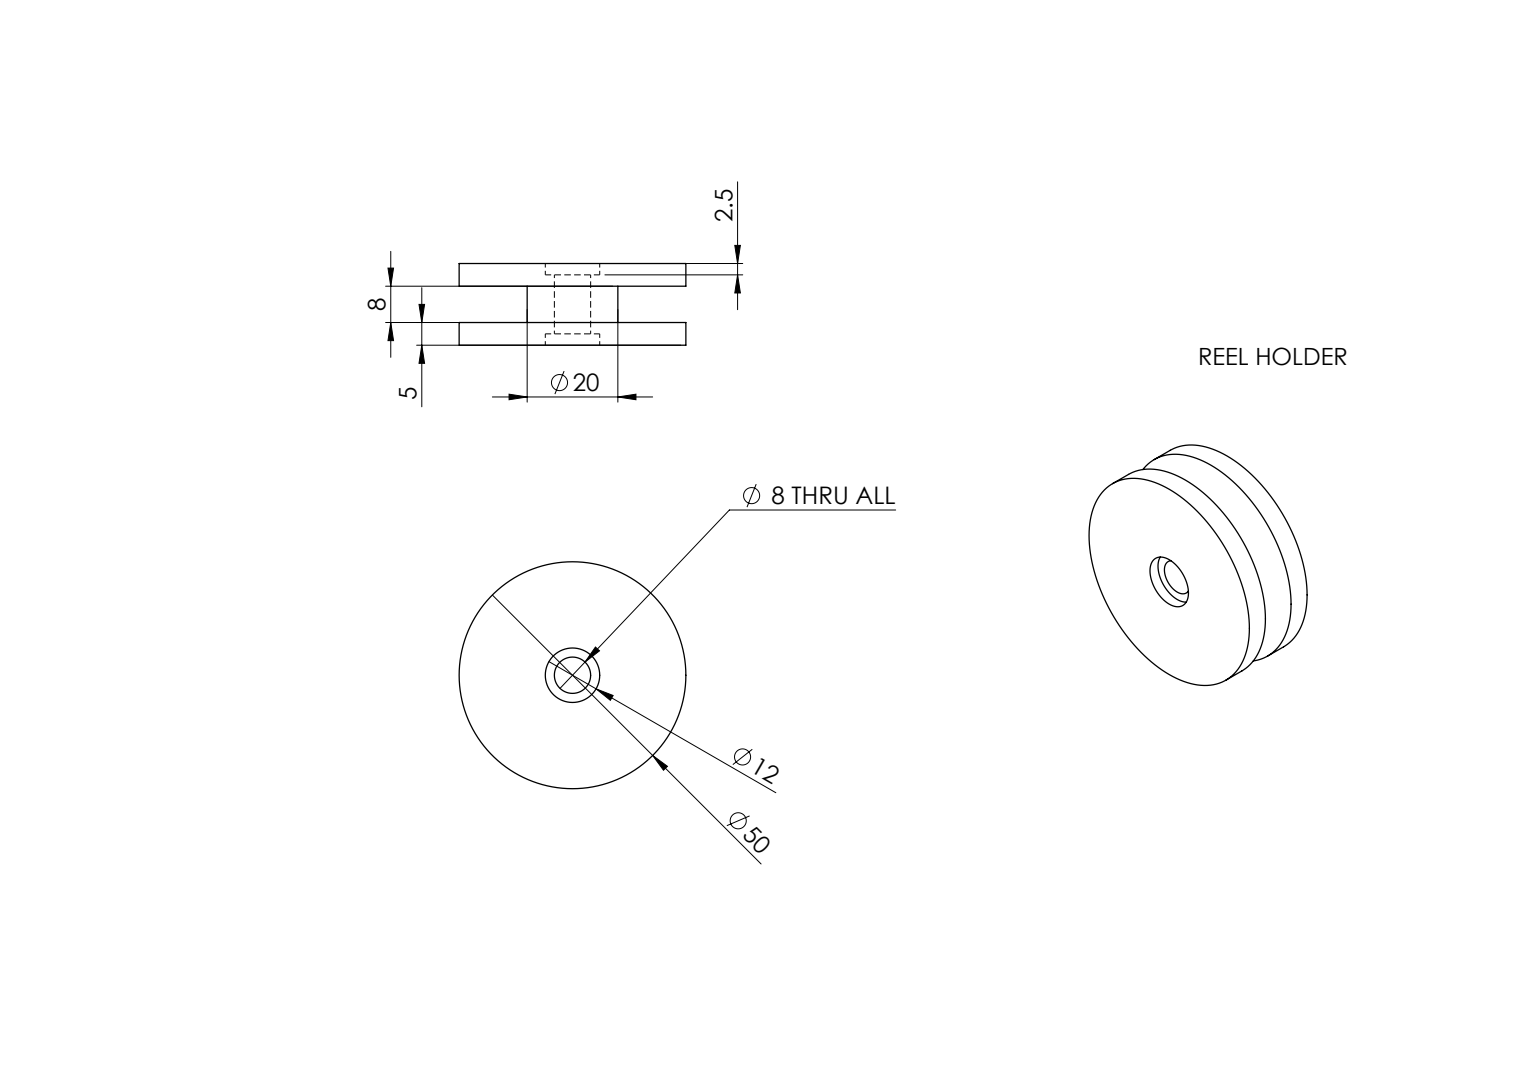
ISO-10303-21;
HEADER;
FILE_DESCRIPTION (('STEP AP214'),
    '1' );
FILE_NAME ('reel holder.step',
    '2026-10-31T03:44:21',
    ( '' ),
    ( '' ),
    'SwSTEP 2.0',
    'SolidWorks 2026',
    '' );
FILE_SCHEMA (( 'AUTOMOTIVE_DESIGN' ));
ENDSEC;

DATA;
#18=EDGE_LOOP ( 'NONE', ( #11625, #15008, #6307, #1224 ) ) ;
#22=AXIS2_PLACEMENT_3D ( 'NONE', #10156, #1151, #17072 ) ;
#37=( NAMED_UNIT ( * ) PLANE_ANGLE_UNIT ( ) SI_UNIT ( $, .RADIAN. ) );
#60=FACE_OUTER_BOUND ( 'NONE', #12914, .T. ) ;
#63=ADVANCED_FACE ( 'NONE', ( #9131 ), #4633, .F. ) ;
#64=ADVANCED_FACE ( 'NONE', ( #5901 ), #7658, .T. ) ;
#74=CIRCLE ( 'NONE', #18561, 24.99999999999999289 ) ;
#181=DIRECTION ( 'NONE',  ( 1.000000000000000000, 0.000000000000000000, 0.000000000000000000 ) ) ;
#266=CYLINDRICAL_SURFACE ( 'NONE', #9428, 5.999999999999977796 ) ;
#280=DIRECTION ( 'NONE',  ( 1.000000000000000000, 0.000000000000000000, 0.000000000000000000 ) ) ;
#318=ADVANCED_FACE ( 'NONE', ( #14500 ), #9696, .T. ) ;
#351=CARTESIAN_POINT ( 'NONE',  ( -154.9999999999999716, -14.99999999999999645, -6.499999999999999112 ) ) ;
#404=EDGE_CURVE ( 'NONE', #12345, #17767, #17395, .T. ) ;
#429=DIRECTION ( 'NONE',  ( -0.000000000000000000, -0.000000000000000000, 1.000000000000000000 ) ) ;
#448=ORIENTED_EDGE ( 'NONE', *, *, #5602, .F. ) ;
#586=CARTESIAN_POINT ( 'NONE',  ( -154.9999999999999716, -14.99999999999999645, 4.000000000000000000 ) ) ;
#587=CIRCLE ( 'NONE', #6229, 5.999999999999977796 ) ;
#601=VECTOR ( 'NONE', #10729, 1000.000000000000000 ) ;
#605=MECHANICAL_DESIGN_GEOMETRIC_PRESENTATION_REPRESENTATION('',(#15624),#12814);
#684=ORIENTED_EDGE ( 'NONE', *, *, #1869, .T. ) ;
#788=AXIS2_PLACEMENT_3D ( 'NONE', #11144, #17151, #5374 ) ;
#800=LINE ( 'NONE', #6771, #1505 ) ;
#861=DIRECTION ( 'NONE',  ( -1.000000000000000000, 0.000000000000000000, 0.000000000000000000 ) ) ;
#869=VERTEX_POINT ( 'NONE', #18994 ) ;
#870=VERTEX_POINT ( 'NONE', #11414 ) ;
#878=DIRECTION ( 'NONE',  ( -1.000000000000000000, 0.000000000000000000, 0.000000000000000000 ) ) ;
#884=DIRECTION ( 'NONE',  ( 1.000000000000000000, 0.000000000000000000, 0.000000000000000000 ) ) ;
#1016=ADVANCED_FACE ( 'NONE', ( #6034, #11998 ), #10619, .T. ) ;
#1038=PRODUCT_DEFINITION_FORMATION_WITH_SPECIFIED_SOURCE ( 'ANY', '', #17923, .NOT_KNOWN. ) ;
#1083=CARTESIAN_POINT ( 'NONE',  ( -154.9999999999999716, -14.99999999999999645, 4.000000000000000000 ) ) ;
#1151=DIRECTION ( 'NONE',  ( 0.000000000000000000, 0.000000000000000000, -1.000000000000000000 ) ) ;
#1224=ORIENTED_EDGE ( 'NONE', *, *, #8355, .F. ) ;
#1418=AXIS2_PLACEMENT_3D ( 'NONE', #5586, #3834, #884 ) ;
#1420=ORIENTED_EDGE ( 'NONE', *, *, #3761, .T. ) ;
#1439=EDGE_LOOP ( 'NONE', ( #2082, #16900, #12486, #14325 ) ) ;
#1454=EDGE_LOOP ( 'NONE', ( #9792, #2037 ) ) ;
#1483=PRODUCT_CONTEXT ( 'NONE', #11764, 'mechanical' ) ;
#1505=VECTOR ( 'NONE', #18753, 1000.000000000000000 ) ;
#1512=EDGE_LOOP ( 'NONE', ( #14590, #15562, #17642, #12838 ) ) ;
#1575=FACE_BOUND ( 'NONE', #7460, .T. ) ;
#1588=VECTOR ( 'NONE', #1817, 1000.000000000000000 ) ;
#1607=AXIS2_PLACEMENT_3D ( 'NONE', #1997, #7773, #4752 ) ;
#1609=PRESENTATION_STYLE_ASSIGNMENT (( #17632 ) ) ;
#1626=DIRECTION ( 'NONE',  ( 1.000000000000000000, 0.000000000000000000, 0.000000000000000000 ) ) ;
#1628=AXIS2_PLACEMENT_3D ( 'NONE', #3357, #15497, #5009 ) ;
#1636=ORIENTED_EDGE ( 'NONE', *, *, #8355, .T. ) ;
#1648=LINE ( 'NONE', #7515, #16648 ) ;
#1796=DIRECTION ( 'NONE',  ( -0.000000000000000000, -0.000000000000000000, 1.000000000000000000 ) ) ;
#1804=CARTESIAN_POINT ( 'NONE',  ( -179.9999999999999716, -15.00000000000000000, -9.000000000000000000 ) ) ;
#1817=DIRECTION ( 'NONE',  ( 0.000000000000000000, 0.000000000000000000, -1.000000000000000000 ) ) ;
#1835=( LENGTH_UNIT ( ) NAMED_UNIT ( * ) SI_UNIT ( .MILLI., .METRE. ) );
#1869=EDGE_CURVE ( 'NONE', #17340, #19190, #16799, .T. ) ;
#1997=CARTESIAN_POINT ( 'NONE',  ( -154.9999999999999716, -14.99999999999999645, -9.000000000000000000 ) ) ;
#2021=AXIS2_PLACEMENT_3D ( 'NONE', #12770, #10013, #11384 ) ;
#2037=ORIENTED_EDGE ( 'NONE', *, *, #13822, .F. ) ;
#2082=ORIENTED_EDGE ( 'NONE', *, *, #11418, .F. ) ;
#2102=CLOSED_SHELL ( 'NONE', ( #4793, #63, #16827, #318, #6766, #9044, #8811, #10108, #5089, #5235, #9436, #64, #16364, #16884, #4440, #2460, #1016, #18165 ) ) ;
#2171=( GEOMETRIC_REPRESENTATION_CONTEXT ( 3 ) GLOBAL_UNCERTAINTY_ASSIGNED_CONTEXT ( ( #4414 ) ) GLOBAL_UNIT_ASSIGNED_CONTEXT ( ( #11985, #15951, #16609 ) ) REPRESENTATION_CONTEXT ( 'NONE', 'WORKASPACE' ) );
#2173=CARTESIAN_POINT ( 'NONE',  ( -154.9999999999999716, -14.99999999999999645, 9.000000000000000000 ) ) ;
#2233=CIRCLE ( 'NONE', #4098, 5.999999999999977796 ) ;
#2309=ORIENTED_EDGE ( 'NONE', *, *, #9763, .F. ) ;
#2327=CIRCLE ( 'NONE', #4523, 24.99999999999999289 ) ;
#2420=VERTEX_POINT ( 'NONE', #9185 ) ;
#2460=ADVANCED_FACE ( 'NONE', ( #6430 ), #266, .F. ) ;
#2472=DIRECTION ( 'NONE',  ( -1.000000000000000000, 0.000000000000000000, 0.000000000000000000 ) ) ;
#2502=DIRECTION ( 'NONE',  ( 1.000000000000000000, 0.000000000000000000, -0.000000000000000000 ) ) ;
#2538=VERTEX_POINT ( 'NONE', #14440 ) ;
#2542=DIRECTION ( 'NONE',  ( 0.000000000000000000, 0.000000000000000000, 1.000000000000000000 ) ) ;
#2544=ORIENTED_EDGE ( 'NONE', *, *, #10861, .T. ) ;
#2576=CIRCLE ( 'NONE', #1628, 10.00000000000000888 ) ;
#2636=SURFACE_SIDE_STYLE ('',( #15030 ) ) ;
#2693=PLANE ( 'NONE',  #16419 ) ;
#2722=AXIS2_PLACEMENT_3D ( 'NONE', #2861, #11750, #13233 ) ;
#2816=EDGE_CURVE ( 'NONE', #19190, #17340, #74, .T. ) ;
#2861=CARTESIAN_POINT ( 'NONE',  ( -154.9999999999999716, -14.99999999999999645, 9.000000000000000000 ) ) ;
#2871=CARTESIAN_POINT ( 'NONE',  ( 0.000000000000000000, 0.000000000000000000, 0.000000000000000000 ) ) ;
#2872=EDGE_CURVE ( 'NONE', #7670, #17070, #14138, .T. ) ;
#2989=CARTESIAN_POINT ( 'NONE',  ( -154.9999999999999716, -14.99999999999999645, -9.000000000000000000 ) ) ;
#3030=VERTEX_POINT ( 'NONE', #7423 ) ;
#3069=AXIS2_PLACEMENT_3D ( 'NONE', #10990, #3551, #16996 ) ;
#3073=STYLED_ITEM('',(#19461),#8428);
#3119=CARTESIAN_POINT ( 'NONE',  ( -160.9999999999999432, -14.99999999999999645, -6.499999999999999112 ) ) ;
#3161=CIRCLE ( 'NONE', #10321, 4.000000000000003553 ) ;
#3180=CIRCLE ( 'NONE', #1607, 5.999999999999977796 ) ;
#3357=CARTESIAN_POINT ( 'NONE',  ( -154.9999999999999716, -14.99999999999999645, 4.000000000000000000 ) ) ;
#3366=CARTESIAN_POINT ( 'NONE',  ( -158.9999999999999716, -14.99999999999999645, 15.00000000000000000 ) ) ;
#3393=VERTEX_POINT ( 'NONE', #6121 ) ;
#3476=PLANE ( 'NONE',  #12019 ) ;
#3551=DIRECTION ( 'NONE',  ( -0.000000000000000000, -0.000000000000000000, 1.000000000000000000 ) ) ;
#3652=LINE ( 'NONE', #3366, #18836 ) ;
#3761=EDGE_CURVE ( 'NONE', #17070, #7670, #11391, .T. ) ;
#3792=EDGE_CURVE ( 'NONE', #8294, #12345, #18966, .T. ) ;
#3834=DIRECTION ( 'NONE',  ( -0.000000000000000000, -0.000000000000000000, 1.000000000000000000 ) ) ;
#3923=VERTEX_POINT ( 'NONE', #7566 ) ;
#3952=CARTESIAN_POINT ( 'NONE',  ( -129.9999999999999716, -14.99999999999999645, -3.999999999999999112 ) ) ;
#4000=CIRCLE ( 'NONE', #12439, 4.000000000000003553 ) ;
#4005=CARTESIAN_POINT ( 'NONE',  ( -160.9999999999999432, -14.99999999999999645, 9.000000000000000000 ) ) ;
#4010=ORIENTED_EDGE ( 'NONE', *, *, #7307, .F. ) ;
#4018=EDGE_CURVE ( 'NONE', #4718, #4669, #18635, .T. ) ;
#4042=DIRECTION ( 'NONE',  ( 1.000000000000000000, 0.000000000000000000, 0.000000000000000000 ) ) ;
#4098=AXIS2_PLACEMENT_3D ( 'NONE', #2989, #16516, #5825 ) ;
#4160=DIRECTION ( 'NONE',  ( 1.000000000000000000, 0.000000000000000000, 0.000000000000000000 ) ) ;
#4180=DIRECTION ( 'NONE',  ( 1.000000000000000000, 0.000000000000000000, 0.000000000000000000 ) ) ;
#4185=ORIENTED_EDGE ( 'NONE', *, *, #6921, .T. ) ;
#4252=ORIENTED_EDGE ( 'NONE', *, *, #5602, .T. ) ;
#4344=ORIENTED_EDGE ( 'NONE', *, *, #14162, .F. ) ;
#4374=CIRCLE ( 'NONE', #15323, 4.000000000000003553 ) ;
#4414=UNCERTAINTY_MEASURE_WITH_UNIT (LENGTH_MEASURE( 1.000000000000000082E-05 ), #11985, 'distance_accuracy_value', 'NONE');
#4428=DIRECTION ( 'NONE',  ( 0.000000000000000000, 0.000000000000000000, -1.000000000000000000 ) ) ;
#4429=CARTESIAN_POINT ( 'NONE',  ( -150.9999999999999716, -14.99999999999999645, 15.00000000000000000 ) ) ;
#4437=FACE_OUTER_BOUND ( 'NONE', #17799, .T. ) ;
#4440=ADVANCED_FACE ( 'NONE', ( #19342, #1575 ), #5884, .T. ) ;
#4474=ORIENTED_EDGE ( 'NONE', *, *, #13822, .T. ) ;
#4475=DIRECTION ( 'NONE',  ( 0.000000000000000000, 0.000000000000000000, 1.000000000000000000 ) ) ;
#4495=CARTESIAN_POINT ( 'NONE',  ( -129.9999999999999716, -14.99999999999999645, -3.999999999999999112 ) ) ;
#4523=AXIS2_PLACEMENT_3D ( 'NONE', #13255, #9818, #8558 ) ;
#4534=AXIS2_PLACEMENT_3D ( 'NONE', #2173, #15305, #18460 ) ;
#4562=DIRECTION ( 'NONE',  ( 0.000000000000000000, 0.000000000000000000, -1.000000000000000000 ) ) ;
#4563=DIRECTION ( 'NONE',  ( -0.000000000000000000, -0.000000000000000000, 1.000000000000000000 ) ) ;
#4567=CARTESIAN_POINT ( 'NONE',  ( -179.9999999999999716, -14.99999999999999289, 3.999999999999999112 ) ) ;
#4633=CYLINDRICAL_SURFACE ( 'NONE', #16829, 5.999999999999977796 ) ;
#4669=VERTEX_POINT ( 'NONE', #4005 ) ;
#4689=( NAMED_UNIT ( * ) SI_UNIT ( $, .STERADIAN. ) SOLID_ANGLE_UNIT ( ) );
#4703=AXIS2_PLACEMENT_3D ( 'NONE', #16401, #14611, #4042 ) ;
#4718=VERTEX_POINT ( 'NONE', #5273 ) ;
#4752=DIRECTION ( 'NONE',  ( 1.000000000000000000, 0.000000000000000000, 0.000000000000000000 ) ) ;
#4755=DIRECTION ( 'NONE',  ( 0.000000000000000000, 0.000000000000000000, -1.000000000000000000 ) ) ;
#4759=FACE_OUTER_BOUND ( 'NONE', #18, .T. ) ;
#4783=DIRECTION ( 'NONE',  ( 1.000000000000000000, 0.000000000000000000, 0.000000000000000000 ) ) ;
#4793=ADVANCED_FACE ( 'NONE', ( #11346 ), #5172, .F. ) ;
#4852=DIRECTION ( 'NONE',  ( -0.000000000000000000, -0.000000000000000000, 1.000000000000000000 ) ) ;
#4874=CARTESIAN_POINT ( 'NONE',  ( -154.9999999999999716, -14.99999999999999645, 6.499999999999999112 ) ) ;
#4952=VERTEX_POINT ( 'NONE', #19224 ) ;
#4966=CIRCLE ( 'NONE', #10293, 10.00000000000000888 ) ;
#5009=DIRECTION ( 'NONE',  ( 1.000000000000000000, 0.000000000000000000, 0.000000000000000000 ) ) ;
#5089=ADVANCED_FACE ( 'NONE', ( #6691, #12773 ), #3476, .F. ) ;
#5172=CYLINDRICAL_SURFACE ( 'NONE', #788, 5.999999999999977796 ) ;
#5216=AXIS2_PLACEMENT_3D ( 'NONE', #18382, #429, #10898 ) ;
#5235=ADVANCED_FACE ( 'NONE', ( #19271, #5510 ), #2693, .T. ) ;
#5254=ORIENTED_EDGE ( 'NONE', *, *, #5301, .T. ) ;
#5262=CARTESIAN_POINT ( 'NONE',  ( -154.9999999999999716, -14.99999999999999645, 9.000000000000000000 ) ) ;
#5273=CARTESIAN_POINT ( 'NONE',  ( -149.0000000000000000, -14.99999999999999645, 9.000000000000000000 ) ) ;
#5298=CIRCLE ( 'NONE', #6245, 5.999999999999977796 ) ;
#5301=EDGE_CURVE ( 'NONE', #16254, #8294, #2327, .T. ) ;
#5313=CARTESIAN_POINT ( 'NONE',  ( -129.9999999999999716, -14.99999999999999645, -9.000000000000000000 ) ) ;
#5320=DIRECTION ( 'NONE',  ( 1.000000000000000000, 0.000000000000000000, -0.000000000000000000 ) ) ;
#5374=DIRECTION ( 'NONE',  ( 1.000000000000000000, 0.000000000000000000, 0.000000000000000000 ) ) ;
#5510=FACE_OUTER_BOUND ( 'NONE', #8020, .T. ) ;
#5545=EDGE_CURVE ( 'NONE', #869, #3393, #10306, .T. ) ;
#5586=CARTESIAN_POINT ( 'NONE',  ( -154.9999999999999716, -14.99999999999999645, -9.000000000000000000 ) ) ;
#5602=EDGE_CURVE ( 'NONE', #869, #10775, #2576, .T. ) ;
#5647=CARTESIAN_POINT ( 'NONE',  ( -154.9999999999999716, -14.99999999999999645, 6.499999999999999112 ) ) ;
#5655=FACE_OUTER_BOUND ( 'NONE', #5723, .T. ) ;
#5661=DIRECTION ( 'NONE',  ( 1.000000000000000000, 0.000000000000000000, 0.000000000000000000 ) ) ;
#5675=AXIS2_PLACEMENT_3D ( 'NONE', #10237, #12002, #16238 ) ;
#5706=DIRECTION ( 'NONE',  ( 1.000000000000000000, 0.000000000000000000, 0.000000000000000000 ) ) ;
#5710=FACE_BOUND ( 'NONE', #1454, .T. ) ;
#5723=EDGE_LOOP ( 'NONE', ( #14570, #18536, #6745, #15319 ) ) ;
#5782=UNCERTAINTY_MEASURE_WITH_UNIT (LENGTH_MEASURE( 1.000000000000000082E-05 ), #1835, 'distance_accuracy_value', 'NONE');
#5825=DIRECTION ( 'NONE',  ( 1.000000000000000000, 0.000000000000000000, 0.000000000000000000 ) ) ;
#5864=EDGE_LOOP ( 'NONE', ( #9344, #6932, #10169, #7931 ) ) ;
#5884=PLANE ( 'NONE',  #10782 ) ;
#5901=FACE_OUTER_BOUND ( 'NONE', #18988, .T. ) ;
#5998=VECTOR ( 'NONE', #19401, 1000.000000000000000 ) ;
#6034=FACE_OUTER_BOUND ( 'NONE', #9664, .T. ) ;
#6113=CIRCLE ( 'NONE', #11103, 10.00000000000000888 ) ;
#6121=CARTESIAN_POINT ( 'NONE',  ( -144.9999999999999716, -14.99999999999999467, -4.000000000000000000 ) ) ;
#6229=AXIS2_PLACEMENT_3D ( 'NONE', #5262, #2542, #8204 ) ;
#6238=ORIENTED_EDGE ( 'NONE', *, *, #17697, .T. ) ;
#6245=AXIS2_PLACEMENT_3D ( 'NONE', #5647, #4475, #4180 ) ;
#6251=DIRECTION ( 'NONE',  ( 0.000000000000000000, 0.000000000000000000, 1.000000000000000000 ) ) ;
#6264=PRODUCT_DEFINITION ( 'UNKNOWN', '', #1038, #9291 ) ;
#6307=ORIENTED_EDGE ( 'NONE', *, *, #7307, .T. ) ;
#6428=DIRECTION ( 'NONE',  ( 1.000000000000000000, 0.000000000000000000, 0.000000000000000000 ) ) ;
#6430=FACE_OUTER_BOUND ( 'NONE', #16684, .T. ) ;
#6436=AXIS2_PLACEMENT_3D ( 'NONE', #12043, #7630, #280 ) ;
#6458=ORIENTED_EDGE ( 'NONE', *, *, #404, .F. ) ;
#6481=VECTOR ( 'NONE', #6846, 1000.000000000000000 ) ;
#6500=DIRECTION ( 'NONE',  ( -1.000000000000000000, 0.000000000000000000, 0.000000000000000000 ) ) ;
#6560=FACE_OUTER_BOUND ( 'NONE', #1512, .T. ) ;
#6662=DIRECTION ( 'NONE',  ( -0.000000000000000000, -0.000000000000000000, -1.000000000000000000 ) ) ;
#6691=FACE_BOUND ( 'NONE', #6831, .T. ) ;
#6745=ORIENTED_EDGE ( 'NONE', *, *, #19262, .T. ) ;
#6755=DIRECTION ( 'NONE',  ( 1.000000000000000000, 0.000000000000000000, 0.000000000000000000 ) ) ;
#6766=ADVANCED_FACE ( 'NONE', ( #60 ), #17714, .T. ) ;
#6771=CARTESIAN_POINT ( 'NONE',  ( -164.9999999999999716, -14.99999999999999645, 4.000000000000000000 ) ) ;
#6805=ORIENTED_EDGE ( 'NONE', *, *, #9511, .T. ) ;
#6831=EDGE_LOOP ( 'NONE', ( #15973, #4252 ) ) ;
#6846=DIRECTION ( 'NONE',  ( -0.000000000000000000, -0.000000000000000000, 1.000000000000000000 ) ) ;
#6921=EDGE_CURVE ( 'NONE', #7670, #19190, #13379, .T. ) ;
#6932=ORIENTED_EDGE ( 'NONE', *, *, #2872, .T. ) ;
#7024=ORIENTED_EDGE ( 'NONE', *, *, #9763, .T. ) ;
#7170=CARTESIAN_POINT ( 'NONE',  ( -154.9999999999999716, -14.99999999999999645, 4.000000000000000000 ) ) ;
#7187=VERTEX_POINT ( 'NONE', #11487 ) ;
#7190=ORIENTED_EDGE ( 'NONE', *, *, #3761, .F. ) ;
#7213=AXIS2_PLACEMENT_3D ( 'NONE', #13647, #1796, #14017 ) ;
#7298=ORIENTED_EDGE ( 'NONE', *, *, #15386, .T. ) ;
#7307=EDGE_CURVE ( 'NONE', #7187, #9732, #14906, .T. ) ;
#7355=AXIS2_PLACEMENT_3D ( 'NONE', #10428, #4563, #16718 ) ;
#7365=AXIS2_PLACEMENT_3D ( 'NONE', #1083, #12649, #2472 ) ;
#7423=CARTESIAN_POINT ( 'NONE',  ( -160.9999999999999432, -14.99999999999999645, -9.000000000000000000 ) ) ;
#7434=ORIENTED_EDGE ( 'NONE', *, *, #12646, .F. ) ;
#7440=( GEOMETRIC_REPRESENTATION_CONTEXT ( 3 ) GLOBAL_UNCERTAINTY_ASSIGNED_CONTEXT ( ( #5782 ) ) GLOBAL_UNIT_ASSIGNED_CONTEXT ( ( #1835, #18126, #4689 ) ) REPRESENTATION_CONTEXT ( 'NONE', 'WORKASPACE' ) );
#7460=EDGE_LOOP ( 'NONE', ( #11837, #1636 ) ) ;
#7486=EDGE_CURVE ( 'NONE', #2420, #11109, #13567, .T. ) ;
#7515=CARTESIAN_POINT ( 'NONE',  ( -160.9999999999999432, -14.99999999999999645, -6.499999999999999112 ) ) ;
#7564=CARTESIAN_POINT ( 'NONE',  ( -129.9999999999999716, -14.99999999999999645, 3.999999999999999112 ) ) ;
#7566=CARTESIAN_POINT ( 'NONE',  ( -149.0000000000000000, -14.99999999999999645, 6.499999999999999112 ) ) ;
#7576=( LENGTH_UNIT ( ) NAMED_UNIT ( * ) SI_UNIT ( .MILLI., .METRE. ) );
#7598=EDGE_CURVE ( 'NONE', #8294, #16254, #8336, .T. ) ;
#7613=DIRECTION ( 'NONE',  ( 1.000000000000000000, 0.000000000000000000, 0.000000000000000000 ) ) ;
#7630=DIRECTION ( 'NONE',  ( -0.000000000000000000, -0.000000000000000000, 1.000000000000000000 ) ) ;
#7658=CYLINDRICAL_SURFACE ( 'NONE', #13051, 24.99999999999999289 ) ;
#7670=VERTEX_POINT ( 'NONE', #11187 ) ;
#7773=DIRECTION ( 'NONE',  ( -0.000000000000000000, -0.000000000000000000, 1.000000000000000000 ) ) ;
#7931=ORIENTED_EDGE ( 'NONE', *, *, #2816, .F. ) ;
#7953=VECTOR ( 'NONE', #15911, 1000.000000000000000 ) ;
#8020=EDGE_LOOP ( 'NONE', ( #684, #16341 ) ) ;
#8132=DIRECTION ( 'NONE',  ( 0.000000000000000000, 0.000000000000000000, 1.000000000000000000 ) ) ;
#8204=DIRECTION ( 'NONE',  ( 1.000000000000000000, 0.000000000000000000, 0.000000000000000000 ) ) ;
#8226=CARTESIAN_POINT ( 'NONE',  ( -154.9999999999999716, -14.99999999999999645, -9.000000000000000000 ) ) ;
#8294=VERTEX_POINT ( 'NONE', #4495 ) ;
#8319=CARTESIAN_POINT ( 'NONE',  ( -154.9999999999999716, -14.99999999999999645, 6.499999999999999112 ) ) ;
#8336=CIRCLE ( 'NONE', #5216, 24.99999999999999289 ) ;
#8355=EDGE_CURVE ( 'NONE', #4952, #9732, #4000, .T. ) ;
#8394=DIRECTION ( 'NONE',  ( 1.000000000000000000, 0.000000000000000000, 0.000000000000000000 ) ) ;
#8428=MANIFOLD_SOLID_BREP ( 'Mirror3', #2102 ) ;
#8503=ORIENTED_EDGE ( 'NONE', *, *, #18760, .F. ) ;
#8558=DIRECTION ( 'NONE',  ( 1.000000000000000000, 0.000000000000000000, 0.000000000000000000 ) ) ;
#8589=FILL_AREA_STYLE ('',( #9041 ) ) ;
#8595=CARTESIAN_POINT ( 'NONE',  ( -154.9999999999999716, -14.99999999999999645, 3.999999999999999112 ) ) ;
#8665=SHAPE_REPRESENTATION ( 'reel holder', ( #10359 ), #2171 ) ;
#8794=ORIENTED_EDGE ( 'NONE', *, *, #2872, .F. ) ;
#8811=ADVANCED_FACE ( 'NONE', ( #4759 ), #10720, .F. ) ;
#8834=DIRECTION ( 'NONE',  ( 0.000000000000000000, 0.000000000000000000, 1.000000000000000000 ) ) ;
#8842=DIRECTION ( 'NONE',  ( -0.000000000000000000, -0.000000000000000000, 1.000000000000000000 ) ) ;
#8856=DIRECTION ( 'NONE',  ( -0.000000000000000000, -0.000000000000000000, -1.000000000000000000 ) ) ;
#8996=CIRCLE ( 'NONE', #3069, 5.999999999999977796 ) ;
#9017=SHAPE_DEFINITION_REPRESENTATION ( #19343, #8665 ) ;
#9041=FILL_AREA_STYLE_COLOUR ( '', #17203 ) ;
#9044=ADVANCED_FACE ( 'NONE', ( #17185 ), #17383, .F. ) ;
#9113=DIRECTION ( 'NONE',  ( 1.000000000000000000, 0.000000000000000000, -0.000000000000000000 ) ) ;
#9131=FACE_OUTER_BOUND ( 'NONE', #15370, .T. ) ;
#9148=EDGE_CURVE ( 'NONE', #10775, #869, #6113, .T. ) ;
#9170=CARTESIAN_POINT ( 'NONE',  ( -154.9999999999999716, -14.99999999999999645, 15.00000000000000000 ) ) ;
#9185=CARTESIAN_POINT ( 'NONE',  ( -149.0000000000000000, -14.99999999999999645, -6.499999999999999112 ) ) ;
#9223=CARTESIAN_POINT ( 'NONE',  ( -144.9999999999999716, -14.99999999999999467, 4.000000000000000000 ) ) ;
#9291=PRODUCT_DEFINITION_CONTEXT ( 'detailed design', #18441, 'design' ) ;
#9344=ORIENTED_EDGE ( 'NONE', *, *, #6921, .F. ) ;
#9428=AXIS2_PLACEMENT_3D ( 'NONE', #13786, #12222, #4783 ) ;
#9436=ADVANCED_FACE ( 'NONE', ( #6560 ), #15586, .T. ) ;
#9494=ORIENTED_EDGE ( 'NONE', *, *, #404, .T. ) ;
#9511=EDGE_CURVE ( 'NONE', #3923, #2538, #10182, .T. ) ;
#9575=DIRECTION ( 'NONE',  ( -0.000000000000000000, -0.000000000000000000, 1.000000000000000000 ) ) ;
#9608=DIRECTION ( 'NONE',  ( 1.000000000000000000, 0.000000000000000000, 0.000000000000000000 ) ) ;
#9659=CIRCLE ( 'NONE', #14677, 10.00000000000000888 ) ;
#9664=EDGE_LOOP ( 'NONE', ( #2309, #7434 ) ) ;
#9691=FACE_BOUND ( 'NONE', #11497, .T. ) ;
#9696=CYLINDRICAL_SURFACE ( 'NONE', #7365, 10.00000000000000888 ) ;
#9724=CARTESIAN_POINT ( 'NONE',  ( -154.9999999999999716, -14.99999999999999645, 3.999999999999999112 ) ) ;
#9732=VERTEX_POINT ( 'NONE', #16082 ) ;
#9736=EDGE_LOOP ( 'NONE', ( #7190, #8794 ) ) ;
#9763=EDGE_CURVE ( 'NONE', #2420, #11339, #16784, .T. ) ;
#9792=ORIENTED_EDGE ( 'NONE', *, *, #13722, .F. ) ;
#9818=DIRECTION ( 'NONE',  ( -0.000000000000000000, -0.000000000000000000, 1.000000000000000000 ) ) ;
#9917=DIRECTION ( 'NONE',  ( 0.000000000000000000, 0.000000000000000000, 1.000000000000000000 ) ) ;
#9999=LINE ( 'NONE', #19156, #12829 ) ;
#10013=DIRECTION ( 'NONE',  ( 0.000000000000000000, 0.000000000000000000, 1.000000000000000000 ) ) ;
#10033=CARTESIAN_POINT ( 'NONE',  ( -164.9999999999999716, -14.99999999999999645, 4.000000000000000000 ) ) ;
#10037=EDGE_LOOP ( 'NONE', ( #7024, #15755, #16509, #14469 ) ) ;
#10076=AXIS2_PLACEMENT_3D ( 'NONE', #13299, #15251, #7613 ) ;
#10108=ADVANCED_FACE ( 'NONE', ( #14272 ), #17535, .T. ) ;
#10155=DIRECTION ( 'NONE',  ( 0.000000000000000000, 0.000000000000000000, 1.000000000000000000 ) ) ;
#10156=CARTESIAN_POINT ( 'NONE',  ( -154.9999999999999716, -14.99999999999999645, -3.999999999999999112 ) ) ;
#10169=ORIENTED_EDGE ( 'NONE', *, *, #18097, .T. ) ;
#10182=CIRCLE ( 'NONE', #18976, 5.999999999999977796 ) ;
#10237=CARTESIAN_POINT ( 'NONE',  ( -154.9999999999999716, -14.99999999999999645, 3.999999999999999112 ) ) ;
#10293=AXIS2_PLACEMENT_3D ( 'NONE', #13972, #15457, #13880 ) ;
#10306=LINE ( 'NONE', #9223, #11942 ) ;
#10321=AXIS2_PLACEMENT_3D ( 'NONE', #351, #4852, #6500 ) ;
#10330=AXIS2_PLACEMENT_3D ( 'NONE', #8226, #15485, #6755 ) ;
#10359=AXIS2_PLACEMENT_3D ( 'NONE', #2871, #8834, #16191 ) ;
#10401=PLANE ( 'NONE',  #4703 ) ;
#10417=CARTESIAN_POINT ( 'NONE',  ( -164.9999999999999716, -14.99999999999999645, -4.000000000000000000 ) ) ;
#10428=CARTESIAN_POINT ( 'NONE',  ( -154.9999999999999716, -14.99999999999999645, 15.00000000000000000 ) ) ;
#10490=ORIENTED_EDGE ( 'NONE', *, *, #12984, .F. ) ;
#10529=LINE ( 'NONE', #13859, #601 ) ;
#10619=PLANE ( 'NONE',  #13081 ) ;
#10720=CYLINDRICAL_SURFACE ( 'NONE', #7355, 4.000000000000003553 ) ;
#10729=DIRECTION ( 'NONE',  ( -0.000000000000000000, -0.000000000000000000, 1.000000000000000000 ) ) ;
#10733=ORIENTED_EDGE ( 'NONE', *, *, #17722, .T. ) ;
#10775=VERTEX_POINT ( 'NONE', #10033 ) ;
#10782=AXIS2_PLACEMENT_3D ( 'NONE', #16386, #11851, #9113 ) ;
#10861=EDGE_CURVE ( 'NONE', #3030, #11109, #2233, .T. ) ;
#10898=DIRECTION ( 'NONE',  ( 1.000000000000000000, 0.000000000000000000, 0.000000000000000000 ) ) ;
#10951=CARTESIAN_POINT ( 'NONE',  ( -149.0000000000000000, -14.99999999999999645, -9.000000000000000000 ) ) ;
#10990=CARTESIAN_POINT ( 'NONE',  ( -154.9999999999999716, -14.99999999999999645, -6.499999999999999112 ) ) ;
#10992=EDGE_CURVE ( 'NONE', #870, #4952, #3652, .T. ) ;
#10997=DIRECTION ( 'NONE',  ( -0.000000000000000000, -0.000000000000000000, 1.000000000000000000 ) ) ;
#11103=AXIS2_PLACEMENT_3D ( 'NONE', #7170, #17587, #5706 ) ;
#11109=VERTEX_POINT ( 'NONE', #10951 ) ;
#11144=CARTESIAN_POINT ( 'NONE',  ( -154.9999999999999716, -14.99999999999999645, -6.499999999999999112 ) ) ;
#11187=CARTESIAN_POINT ( 'NONE',  ( -179.9999999999999716, -14.99999999999999289, 3.999999999999999112 ) ) ;
#11339=VERTEX_POINT ( 'NONE', #3119 ) ;
#11346=FACE_OUTER_BOUND ( 'NONE', #10037, .T. ) ;
#11384=DIRECTION ( 'NONE',  ( 1.000000000000000000, 0.000000000000000000, 0.000000000000000000 ) ) ;
#11391=CIRCLE ( 'NONE', #2021, 24.99999999999999289 ) ;
#11414=CARTESIAN_POINT ( 'NONE',  ( -158.9999999999999716, -14.99999999999999645, -6.499999999999999112 ) ) ;
#11418=EDGE_CURVE ( 'NONE', #11339, #3030, #1648, .T. ) ;
#11487=CARTESIAN_POINT ( 'NONE',  ( -150.9999999999999716, -14.99999999999999645, -6.499999999999999112 ) ) ;
#11497=EDGE_LOOP ( 'NONE', ( #10733, #2544 ) ) ;
#11548=ORIENTED_EDGE ( 'NONE', *, *, #4018, .T. ) ;
#11607=AXIS2_PLACEMENT_3D ( 'NONE', #18340, #9575, #861 ) ;
#11625=ORIENTED_EDGE ( 'NONE', *, *, #10992, .F. ) ;
#11750=DIRECTION ( 'NONE',  ( 0.000000000000000000, 0.000000000000000000, 1.000000000000000000 ) ) ;
#11764=APPLICATION_CONTEXT ( 'automotive_design' ) ;
#11837=ORIENTED_EDGE ( 'NONE', *, *, #14592, .T. ) ;
#11851=DIRECTION ( 'NONE',  ( 0.000000000000000000, 0.000000000000000000, 1.000000000000000000 ) ) ;
#11857=CARTESIAN_POINT ( 'NONE',  ( -154.9999999999999716, -14.99999999999999645, -6.499999999999999112 ) ) ;
#11942=VECTOR ( 'NONE', #16313, 1000.000000000000000 ) ;
#11974=CARTESIAN_POINT ( 'NONE',  ( -154.9999999999999716, -14.99999999999999645, 6.499999999999999112 ) ) ;
#11985=( LENGTH_UNIT ( ) NAMED_UNIT ( * ) SI_UNIT ( .MILLI., .METRE. ) );
#11998=FACE_BOUND ( 'NONE', #13148, .T. ) ;
#12002=DIRECTION ( 'NONE',  ( 0.000000000000000000, 0.000000000000000000, 1.000000000000000000 ) ) ;
#12005=ORIENTED_EDGE ( 'NONE', *, *, #12504, .F. ) ;
#12016=DIRECTION ( 'NONE',  ( 0.000000000000000000, 0.000000000000000000, -1.000000000000000000 ) ) ;
#12019=AXIS2_PLACEMENT_3D ( 'NONE', #9724, #18775, #5320 ) ;
#12043=CARTESIAN_POINT ( 'NONE',  ( -154.9999999999999716, -14.99999999999999645, -6.499999999999999112 ) ) ;
#12197=LINE ( 'NONE', #13667, #1588 ) ;
#12222=DIRECTION ( 'NONE',  ( -0.000000000000000000, -0.000000000000000000, 1.000000000000000000 ) ) ;
#12345=VERTEX_POINT ( 'NONE', #5313 ) ;
#12439=AXIS2_PLACEMENT_3D ( 'NONE', #4874, #16552, #6428 ) ;
#12486=ORIENTED_EDGE ( 'NONE', *, *, #7486, .T. ) ;
#12504=EDGE_CURVE ( 'NONE', #2538, #4669, #18935, .T. ) ;
#12546=DIRECTION ( 'NONE',  ( 1.000000000000000000, 0.000000000000000000, 0.000000000000000000 ) ) ;
#12646=EDGE_CURVE ( 'NONE', #11339, #2420, #8996, .T. ) ;
#12649=DIRECTION ( 'NONE',  ( -0.000000000000000000, -0.000000000000000000, -1.000000000000000000 ) ) ;
#12770=CARTESIAN_POINT ( 'NONE',  ( -154.9999999999999716, -14.99999999999999645, 3.999999999999999112 ) ) ;
#12773=FACE_OUTER_BOUND ( 'NONE', #9736, .T. ) ;
#12814=( GEOMETRIC_REPRESENTATION_CONTEXT ( 3 ) GLOBAL_UNCERTAINTY_ASSIGNED_CONTEXT ( ( #16573 ) ) GLOBAL_UNIT_ASSIGNED_CONTEXT ( ( #7576, #37, #13558 ) ) REPRESENTATION_CONTEXT ( 'NONE', 'WORKASPACE' ) );
#12829=VECTOR ( 'NONE', #15997, 1000.000000000000000 ) ;
#12838=ORIENTED_EDGE ( 'NONE', *, *, #13722, .T. ) ;
#12914=EDGE_LOOP ( 'NONE', ( #1420, #4185, #13658, #17271 ) ) ;
#12961=CARTESIAN_POINT ( 'NONE',  ( -154.9999999999999716, -14.99999999999999645, 9.000000000000000000 ) ) ;
#12984=EDGE_CURVE ( 'NONE', #10775, #16015, #800, .T. ) ;
#13044=CYLINDRICAL_SURFACE ( 'NONE', #16283, 5.999999999999977796 ) ;
#13051=AXIS2_PLACEMENT_3D ( 'NONE', #13638, #17978, #19266 ) ;
#13081=AXIS2_PLACEMENT_3D ( 'NONE', #18002, #4562, #1626 ) ;
#13104=FACE_OUTER_BOUND ( 'NONE', #15291, .T. ) ;
#13148=EDGE_LOOP ( 'NONE', ( #19416, #6238 ) ) ;
#13233=DIRECTION ( 'NONE',  ( 1.000000000000000000, 0.000000000000000000, 0.000000000000000000 ) ) ;
#13255=CARTESIAN_POINT ( 'NONE',  ( -154.9999999999999716, -14.99999999999999645, -3.999999999999999112 ) ) ;
#13286=ORIENTED_EDGE ( 'NONE', *, *, #7598, .T. ) ;
#13299=CARTESIAN_POINT ( 'NONE',  ( -154.9999999999999716, -14.99999999999999645, 3.999999999999999112 ) ) ;
#13379=LINE ( 'NONE', #4567, #5998 ) ;
#13558=( NAMED_UNIT ( * ) SI_UNIT ( $, .STERADIAN. ) SOLID_ANGLE_UNIT ( ) );
#13567=LINE ( 'NONE', #18095, #13968 ) ;
#13638=CARTESIAN_POINT ( 'NONE',  ( -154.9999999999999716, -14.99999999999999645, -3.999999999999999112 ) ) ;
#13647=CARTESIAN_POINT ( 'NONE',  ( -154.9999999999999716, -14.99999999999999645, -9.000000000000000000 ) ) ;
#13658=ORIENTED_EDGE ( 'NONE', *, *, #1869, .F. ) ;
#13667=CARTESIAN_POINT ( 'NONE',  ( -179.9999999999999716, -15.00000000000000000, -3.999999999999999112 ) ) ;
#13722=EDGE_CURVE ( 'NONE', #16015, #3393, #4966, .T. ) ;
#13786=CARTESIAN_POINT ( 'NONE',  ( -154.9999999999999716, -14.99999999999999645, 6.499999999999999112 ) ) ;
#13799=EDGE_LOOP ( 'NONE', ( #448, #19384, #4474, #10490 ) ) ;
#13822=EDGE_CURVE ( 'NONE', #3393, #16015, #9659, .T. ) ;
#13859=CARTESIAN_POINT ( 'NONE',  ( -149.0000000000000000, -14.99999999999999645, 6.499999999999999112 ) ) ;
#13880=DIRECTION ( 'NONE',  ( 1.000000000000000000, 0.000000000000000000, 0.000000000000000000 ) ) ;
#13900=EDGE_LOOP ( 'NONE', ( #18381, #15247 ) ) ;
#13968=VECTOR ( 'NONE', #4755, 1000.000000000000000 ) ;
#13972=CARTESIAN_POINT ( 'NONE',  ( -154.9999999999999716, -14.99999999999999645, -4.000000000000000000 ) ) ;
#14017=DIRECTION ( 'NONE',  ( 1.000000000000000000, 0.000000000000000000, 0.000000000000000000 ) ) ;
#14023=CARTESIAN_POINT ( 'NONE',  ( -179.9999999999999716, -15.00000000000000000, -3.999999999999999112 ) ) ;
#14106=CIRCLE ( 'NONE', #11607, 4.000000000000003553 ) ;
#14138=CIRCLE ( 'NONE', #10076, 24.99999999999999289 ) ;
#14152=ORIENTED_EDGE ( 'NONE', *, *, #14162, .T. ) ;
#14162=EDGE_CURVE ( 'NONE', #2538, #3923, #5298, .T. ) ;
#14235=EDGE_CURVE ( 'NONE', #3923, #4718, #10529, .T. ) ;
#14272=FACE_OUTER_BOUND ( 'NONE', #5864, .T. ) ;
#14295=CARTESIAN_POINT ( 'NONE',  ( -160.9999999999999432, -14.99999999999999645, 6.499999999999999112 ) ) ;
#14325=ORIENTED_EDGE ( 'NONE', *, *, #10861, .F. ) ;
#14440=CARTESIAN_POINT ( 'NONE',  ( -160.9999999999999432, -14.99999999999999645, 6.499999999999999112 ) ) ;
#14469=ORIENTED_EDGE ( 'NONE', *, *, #7486, .F. ) ;
#14498=ORIENTED_EDGE ( 'NONE', *, *, #19262, .F. ) ;
#14500=FACE_OUTER_BOUND ( 'NONE', #13799, .T. ) ;
#14570=ORIENTED_EDGE ( 'NONE', *, *, #5301, .F. ) ;
#14590=ORIENTED_EDGE ( 'NONE', *, *, #5545, .F. ) ;
#14592=EDGE_CURVE ( 'NONE', #9732, #4952, #4374, .T. ) ;
#14611=DIRECTION ( 'NONE',  ( 0.000000000000000000, 0.000000000000000000, -1.000000000000000000 ) ) ;
#14677=AXIS2_PLACEMENT_3D ( 'NONE', #16947, #6251, #181 ) ;
#14906=LINE ( 'NONE', #4429, #16807 ) ;
#14948=MECHANICAL_DESIGN_GEOMETRIC_PRESENTATION_REPRESENTATION('',(#3073),#7440);
#15008=ORIENTED_EDGE ( 'NONE', *, *, #18751, .F. ) ;
#15030=SURFACE_STYLE_FILL_AREA ( #8589 ) ;
#15059=ORIENTED_EDGE ( 'NONE', *, *, #9511, .F. ) ;
#15247=ORIENTED_EDGE ( 'NONE', *, *, #15386, .F. ) ;
#15251=DIRECTION ( 'NONE',  ( 0.000000000000000000, 0.000000000000000000, 1.000000000000000000 ) ) ;
#15291=EDGE_LOOP ( 'NONE', ( #6458, #14498 ) ) ;
#15305=DIRECTION ( 'NONE',  ( 0.000000000000000000, 0.000000000000000000, 1.000000000000000000 ) ) ;
#15319=ORIENTED_EDGE ( 'NONE', *, *, #3792, .F. ) ;
#15323=AXIS2_PLACEMENT_3D ( 'NONE', #16320, #8856, #4160 ) ;
#15344=ORIENTED_EDGE ( 'NONE', *, *, #12504, .T. ) ;
#15370=EDGE_LOOP ( 'NONE', ( #4344, #15344, #7298, #16251 ) ) ;
#15375=ORIENTED_EDGE ( 'NONE', *, *, #7598, .F. ) ;
#15386=EDGE_CURVE ( 'NONE', #4669, #4718, #587, .T. ) ;
#15457=DIRECTION ( 'NONE',  ( 0.000000000000000000, 0.000000000000000000, 1.000000000000000000 ) ) ;
#15485=DIRECTION ( 'NONE',  ( 0.000000000000000000, 0.000000000000000000, -1.000000000000000000 ) ) ;
#15497=DIRECTION ( 'NONE',  ( 0.000000000000000000, 0.000000000000000000, 1.000000000000000000 ) ) ;
#15562=ORIENTED_EDGE ( 'NONE', *, *, #9148, .F. ) ;
#15586=CYLINDRICAL_SURFACE ( 'NONE', #17091, 10.00000000000000888 ) ;
#15624=STYLED_ITEM ( 'NONE', ( #1609 ), #18337 ) ;
#15690=PLANE ( 'NONE',  #10330 ) ;
#15710=DIRECTION ( 'NONE',  ( -0.000000000000000000, -0.000000000000000000, 1.000000000000000000 ) ) ;
#15734=ORIENTED_EDGE ( 'NONE', *, *, #14235, .T. ) ;
#15755=ORIENTED_EDGE ( 'NONE', *, *, #11418, .T. ) ;
#15787=DIRECTION ( 'NONE',  ( 0.000000000000000000, 0.000000000000000000, 1.000000000000000000 ) ) ;
#15887=CARTESIAN_POINT ( 'NONE',  ( -129.9999999999999716, -14.99999999999999645, 9.000000000000000000 ) ) ;
#15911=DIRECTION ( 'NONE',  ( 0.000000000000000000, 0.000000000000000000, -1.000000000000000000 ) ) ;
#15951=( NAMED_UNIT ( * ) PLANE_ANGLE_UNIT ( ) SI_UNIT ( $, .RADIAN. ) );
#15973=ORIENTED_EDGE ( 'NONE', *, *, #9148, .T. ) ;
#15997=DIRECTION ( 'NONE',  ( 0.000000000000000000, 0.000000000000000000, 1.000000000000000000 ) ) ;
#16015=VERTEX_POINT ( 'NONE', #10417 ) ;
#16063=ORIENTED_EDGE ( 'NONE', *, *, #14592, .F. ) ;
#16082=CARTESIAN_POINT ( 'NONE',  ( -150.9999999999999716, -14.99999999999999645, 6.499999999999999112 ) ) ;
#16191=DIRECTION ( 'NONE',  ( 1.000000000000000000, 0.000000000000000000, 0.000000000000000000 ) ) ;
#16238=DIRECTION ( 'NONE',  ( 1.000000000000000000, 0.000000000000000000, 0.000000000000000000 ) ) ;
#16251=ORIENTED_EDGE ( 'NONE', *, *, #14235, .F. ) ;
#16254=VERTEX_POINT ( 'NONE', #14023 ) ;
#16283=AXIS2_PLACEMENT_3D ( 'NONE', #11857, #4428, #19052 ) ;
#16294=FACE_OUTER_BOUND ( 'NONE', #1439, .T. ) ;
#16312=CIRCLE ( 'NONE', #7213, 24.99999999999999289 ) ;
#16313=DIRECTION ( 'NONE',  ( -0.000000000000000000, -0.000000000000000000, -1.000000000000000000 ) ) ;
#16320=CARTESIAN_POINT ( 'NONE',  ( -154.9999999999999716, -14.99999999999999645, 6.499999999999999112 ) ) ;
#16341=ORIENTED_EDGE ( 'NONE', *, *, #2816, .T. ) ;
#16364=ADVANCED_FACE ( 'NONE', ( #5710, #4437 ), #10401, .F. ) ;
#16386=CARTESIAN_POINT ( 'NONE',  ( -154.9999999999999716, -14.99999999999999645, 6.499999999999999112 ) ) ;
#16401=CARTESIAN_POINT ( 'NONE',  ( -154.9999999999999716, -14.99999999999999645, -3.999999999999999112 ) ) ;
#16416=SHAPE_REPRESENTATION_RELATIONSHIP ( 'NONE' , 'NONE' ,  #8665, #18337 ) ;
#16419=AXIS2_PLACEMENT_3D ( 'NONE', #12961, #9917, #2502 ) ;
#16509=ORIENTED_EDGE ( 'NONE', *, *, #17722, .F. ) ;
#16516=DIRECTION ( 'NONE',  ( -0.000000000000000000, -0.000000000000000000, 1.000000000000000000 ) ) ;
#16552=DIRECTION ( 'NONE',  ( -0.000000000000000000, -0.000000000000000000, -1.000000000000000000 ) ) ;
#16573=UNCERTAINTY_MEASURE_WITH_UNIT (LENGTH_MEASURE( 1.000000000000000082E-05 ), #7576, 'distance_accuracy_value', 'NONE');
#16582=DIRECTION ( 'NONE',  ( -0.000000000000000000, -0.000000000000000000, 1.000000000000000000 ) ) ;
#16609=( NAMED_UNIT ( * ) SI_UNIT ( $, .STERADIAN. ) SOLID_ANGLE_UNIT ( ) );
#16648=VECTOR ( 'NONE', #12016, 1000.000000000000000 ) ;
#16684=EDGE_LOOP ( 'NONE', ( #12005, #15059, #15734, #11548 ) ) ;
#16718=DIRECTION ( 'NONE',  ( 1.000000000000000000, 0.000000000000000000, 0.000000000000000000 ) ) ;
#16781=ORIENTED_EDGE ( 'NONE', *, *, #3792, .T. ) ;
#16784=CIRCLE ( 'NONE', #6436, 5.999999999999977796 ) ;
#16795=CARTESIAN_POINT ( 'NONE',  ( -179.9999999999999716, -14.99999999999999289, 9.000000000000000000 ) ) ;
#16799=CIRCLE ( 'NONE', #2722, 24.99999999999999289 ) ;
#16807=VECTOR ( 'NONE', #16582, 1000.000000000000000 ) ;
#16827=ADVANCED_FACE ( 'NONE', ( #5655 ), #19114, .T. ) ;
#16829=AXIS2_PLACEMENT_3D ( 'NONE', #11974, #8842, #19366 ) ;
#16884=ADVANCED_FACE ( 'NONE', ( #9691, #13104 ), #15690, .T. ) ;
#16900=ORIENTED_EDGE ( 'NONE', *, *, #12646, .T. ) ;
#16947=CARTESIAN_POINT ( 'NONE',  ( -154.9999999999999716, -14.99999999999999645, -4.000000000000000000 ) ) ;
#16996=DIRECTION ( 'NONE',  ( 1.000000000000000000, 0.000000000000000000, 0.000000000000000000 ) ) ;
#17070=VERTEX_POINT ( 'NONE', #7564 ) ;
#17072=DIRECTION ( 'NONE',  ( 1.000000000000000000, 0.000000000000000000, 0.000000000000000000 ) ) ;
#17091=AXIS2_PLACEMENT_3D ( 'NONE', #586, #6662, #878 ) ;
#17151=DIRECTION ( 'NONE',  ( 0.000000000000000000, 0.000000000000000000, -1.000000000000000000 ) ) ;
#17185=FACE_OUTER_BOUND ( 'NONE', #18496, .T. ) ;
#17203=COLOUR_RGB ( '',0.8941176470588234615, 0.8941176470588234615, 0.8941176470588234615 ) ;
#17271=ORIENTED_EDGE ( 'NONE', *, *, #18097, .F. ) ;
#17340=VERTEX_POINT ( 'NONE', #15887 ) ;
#17383=CYLINDRICAL_SURFACE ( 'NONE', #17386, 4.000000000000003553 ) ;
#17386=AXIS2_PLACEMENT_3D ( 'NONE', #9170, #15710, #9608 ) ;
#17395=CIRCLE ( 'NONE', #1418, 24.99999999999999289 ) ;
#17535=CYLINDRICAL_SURFACE ( 'NONE', #19326, 24.99999999999999289 ) ;
#17587=DIRECTION ( 'NONE',  ( 0.000000000000000000, 0.000000000000000000, 1.000000000000000000 ) ) ;
#17632=SURFACE_STYLE_USAGE ( .BOTH. , #2636 ) ;
#17642=ORIENTED_EDGE ( 'NONE', *, *, #12984, .T. ) ;
#17697=EDGE_CURVE ( 'NONE', #870, #7187, #14106, .T. ) ;
#17714=CYLINDRICAL_SURFACE ( 'NONE', #5675, 24.99999999999999289 ) ;
#17722=EDGE_CURVE ( 'NONE', #11109, #3030, #3180, .T. ) ;
#17724=ORIENTED_EDGE ( 'NONE', *, *, #10992, .T. ) ;
#17767=VERTEX_POINT ( 'NONE', #1804 ) ;
#17799=EDGE_LOOP ( 'NONE', ( #13286, #5254 ) ) ;
#17923=PRODUCT ( 'reel holder', 'reel holder', '', ( #1483 ) ) ;
#17978=DIRECTION ( 'NONE',  ( 0.000000000000000000, 0.000000000000000000, -1.000000000000000000 ) ) ;
#18002=CARTESIAN_POINT ( 'NONE',  ( -154.9999999999999716, -14.99999999999999645, -6.499999999999999112 ) ) ;
#18095=CARTESIAN_POINT ( 'NONE',  ( -149.0000000000000000, -14.99999999999999645, -6.499999999999999112 ) ) ;
#18097=EDGE_CURVE ( 'NONE', #17070, #17340, #9999, .T. ) ;
#18126=( NAMED_UNIT ( * ) PLANE_ANGLE_UNIT ( ) SI_UNIT ( $, .RADIAN. ) );
#18165=ADVANCED_FACE ( 'NONE', ( #16294 ), #13044, .F. ) ;
#18337=ADVANCED_BREP_SHAPE_REPRESENTATION ( '', ( #8428, #10359 ), #2171 ) ;
#18340=CARTESIAN_POINT ( 'NONE',  ( -154.9999999999999716, -14.99999999999999645, -6.499999999999999112 ) ) ;
#18381=ORIENTED_EDGE ( 'NONE', *, *, #4018, .F. ) ;
#18382=CARTESIAN_POINT ( 'NONE',  ( -154.9999999999999716, -14.99999999999999645, -3.999999999999999112 ) ) ;
#18441=APPLICATION_CONTEXT ( 'automotive_design' ) ;
#18460=DIRECTION ( 'NONE',  ( 1.000000000000000000, 0.000000000000000000, 0.000000000000000000 ) ) ;
#18496=EDGE_LOOP ( 'NONE', ( #19208, #17724, #16063, #4010 ) ) ;
#18536=ORIENTED_EDGE ( 'NONE', *, *, #18760, .T. ) ;
#18561=AXIS2_PLACEMENT_3D ( 'NONE', #19118, #8132, #5661 ) ;
#18635=CIRCLE ( 'NONE', #4534, 5.999999999999977796 ) ;
#18751=EDGE_CURVE ( 'NONE', #7187, #870, #3161, .T. ) ;
#18753=DIRECTION ( 'NONE',  ( -0.000000000000000000, -0.000000000000000000, -1.000000000000000000 ) ) ;
#18760=EDGE_CURVE ( 'NONE', #16254, #17767, #12197, .T. ) ;
#18775=DIRECTION ( 'NONE',  ( 0.000000000000000000, 0.000000000000000000, 1.000000000000000000 ) ) ;
#18836=VECTOR ( 'NONE', #10997, 1000.000000000000000 ) ;
#18896=EDGE_LOOP ( 'NONE', ( #6805, #14152 ) ) ;
#18935=LINE ( 'NONE', #14295, #6481 ) ;
#18966=LINE ( 'NONE', #3952, #7953 ) ;
#18976=AXIS2_PLACEMENT_3D ( 'NONE', #8319, #15787, #12546 ) ;
#18988=EDGE_LOOP ( 'NONE', ( #8503, #15375, #16781, #9494 ) ) ;
#18994=CARTESIAN_POINT ( 'NONE',  ( -144.9999999999999716, -14.99999999999999467, 4.000000000000000000 ) ) ;
#19052=DIRECTION ( 'NONE',  ( 1.000000000000000000, 0.000000000000000000, 0.000000000000000000 ) ) ;
#19114=CYLINDRICAL_SURFACE ( 'NONE', #22, 24.99999999999999289 ) ;
#19118=CARTESIAN_POINT ( 'NONE',  ( -154.9999999999999716, -14.99999999999999645, 9.000000000000000000 ) ) ;
#19156=CARTESIAN_POINT ( 'NONE',  ( -129.9999999999999716, -14.99999999999999645, 3.999999999999999112 ) ) ;
#19190=VERTEX_POINT ( 'NONE', #16795 ) ;
#19208=ORIENTED_EDGE ( 'NONE', *, *, #17697, .F. ) ;
#19224=CARTESIAN_POINT ( 'NONE',  ( -158.9999999999999716, -14.99999999999999645, 6.499999999999999112 ) ) ;
#19262=EDGE_CURVE ( 'NONE', #17767, #12345, #16312, .T. ) ;
#19266=DIRECTION ( 'NONE',  ( 1.000000000000000000, 0.000000000000000000, 0.000000000000000000 ) ) ;
#19271=FACE_BOUND ( 'NONE', #13900, .T. ) ;
#19326=AXIS2_PLACEMENT_3D ( 'NONE', #8595, #10155, #8394 ) ;
#19342=FACE_OUTER_BOUND ( 'NONE', #18896, .T. ) ;
#19343=PRODUCT_DEFINITION_SHAPE ( 'NONE', 'NONE',  #6264 ) ;
#19366=DIRECTION ( 'NONE',  ( 1.000000000000000000, 0.000000000000000000, 0.000000000000000000 ) ) ;
#19384=ORIENTED_EDGE ( 'NONE', *, *, #5545, .T. ) ;
#19401=DIRECTION ( 'NONE',  ( 0.000000000000000000, 0.000000000000000000, 1.000000000000000000 ) ) ;
#19416=ORIENTED_EDGE ( 'NONE', *, *, #18751, .T. ) ;
#19455=COLOUR_RGB('Sky Blue',0.24,0.69,0.87);
#19456=FILL_AREA_STYLE_COLOUR('',#19455);
#19457=FILL_AREA_STYLE('',(#19456));
#19458=SURFACE_STYLE_FILL_AREA(#19457);
#19459=SURFACE_SIDE_STYLE('',(#19458));
#19460=SURFACE_STYLE_USAGE(.BOTH.,#19459);
#19461=PRESENTATION_STYLE_ASSIGNMENT((#19460));
ENDSEC;
END-ISO-10303-21;
